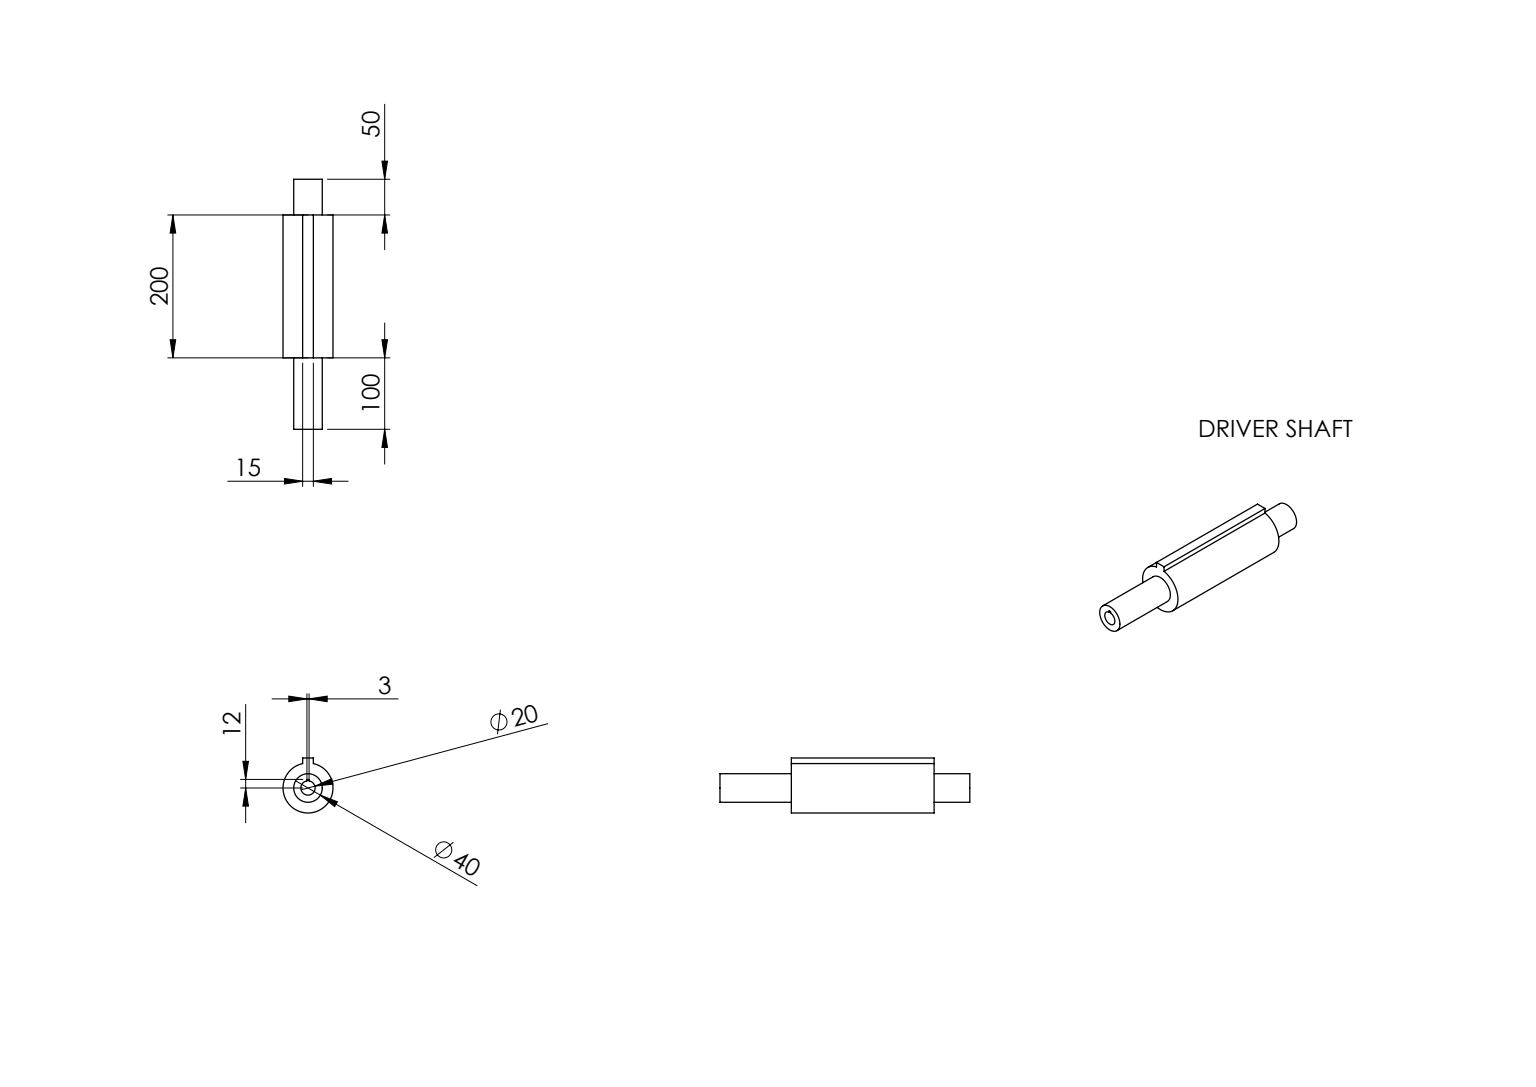
ISO-10303-21;
HEADER;
FILE_DESCRIPTION (('STEP AP214'),
    '1' );
FILE_NAME ('driver shaft.step',
    '2026-10-31T03:46:07',
    ( '' ),
    ( '' ),
    'SwSTEP 2.0',
    'SolidWorks 2026',
    '' );
FILE_SCHEMA (( 'AUTOMOTIVE_DESIGN' ));
ENDSEC;

DATA;
#4=CIRCLE ( 'NONE', #6942, 9.999999999999998224 ) ;
#24=ORIENTED_EDGE ( 'NONE', *, *, #13771, .T. ) ;
#33=DIRECTION ( 'NONE',  ( -1.000000000000000000, -0.000000000000000000, -0.000000000000000000 ) ) ;
#92=DIRECTION ( 'NONE',  ( 1.000000000000000000, 0.000000000000000000, 0.000000000000000000 ) ) ;
#97=ORIENTED_EDGE ( 'NONE', *, *, #11862, .T. ) ;
#125=DIRECTION ( 'NONE',  ( 0.000000000000000000, 0.000000000000000000, 1.000000000000000000 ) ) ;
#141=ORIENTED_EDGE ( 'NONE', *, *, #17752, .T. ) ;
#337=CARTESIAN_POINT ( 'NONE',  ( -2.617478843592795368, -9.739726766683153514, 200.0000120000000265 ) ) ;
#387=LINE ( 'NONE', #18240, #3022 ) ;
#432=CARTESIAN_POINT ( 'NONE',  ( -8.354408924214205001, 5.621797280079010584, 200.0000120000000550 ) ) ;
#474=FACE_OUTER_BOUND ( 'NONE', #7021, .T. ) ;
#545=STYLED_ITEM('',(#23920),#12018);
#550=VERTEX_POINT ( 'NONE', #7568 ) ;
#582=ORIENTED_EDGE ( 'NONE', *, *, #10189, .T. ) ;
#629=VERTEX_POINT ( 'NONE', #2837 ) ;
#663=ORIENTED_EDGE ( 'NONE', *, *, #16433, .T. ) ;
#679=VERTEX_POINT ( 'NONE', #17578 ) ;
#681=CARTESIAN_POINT ( 'NONE',  ( 2.670021022440450587, 9.709363531332249053, 200.0000120000000265 ) ) ;
#699=ORIENTED_EDGE ( 'NONE', *, *, #6704, .F. ) ;
#817=ORIENTED_EDGE ( 'NONE', *, *, #14063, .T. ) ;
#829=VERTEX_POINT ( 'NONE', #1392 ) ;
#869=CARTESIAN_POINT ( 'NONE',  ( -7.499999999999999112, 41.99999999999998579, -100.0000000000000000 ) ) ;
#957=FACE_OUTER_BOUND ( 'NONE', #21689, .T. ) ;
#1000=ORIENTED_EDGE ( 'NONE', *, *, #10407, .F. ) ;
#1015=FACE_OUTER_BOUND ( 'NONE', #12354, .T. ) ;
#1023=VECTOR ( 'NONE', #21634, 1000.000000000000000 ) ;
#1105=DIRECTION ( 'NONE',  ( -0.000000000000000000, -1.000000000000000000, -0.000000000000000000 ) ) ;
#1121=AXIS2_PLACEMENT_3D ( 'NONE', #4909, #12668, #14115 ) ;
#1135=FACE_OUTER_BOUND ( 'NONE', #14500, .T. ) ;
#1144=DIRECTION ( 'NONE',  ( 1.000000000000000000, 0.000000000000000000, 0.000000000000000000 ) ) ;
#1337=ORIENTED_EDGE ( 'NONE', *, *, #20218, .T. ) ;
#1392=CARTESIAN_POINT ( 'NONE',  ( 7.499999999999999112, 41.99999999999998579, -100.0000000000000000 ) ) ;
#1488=CARTESIAN_POINT ( 'NONE',  ( 0.000000000000000000, 0.000000000000000000, 100.0000000000000000 ) ) ;
#1490=DIRECTION ( 'NONE',  ( 0.000000000000000000, -1.000000000000000000, 0.000000000000000000 ) ) ;
#1493=CARTESIAN_POINT ( 'NONE',  ( -7.499999999999999112, 34.18698582794336716, 100.0000000000000000 ) ) ;
#1523=CARTESIAN_POINT ( 'NONE',  ( 0.000000000000000000, 0.000000000000000000, 200.0000119999999981 ) ) ;
#1539=AXIS2_PLACEMENT_3D ( 'NONE', #22452, #8220, #15597 ) ;
#1555=FACE_BOUND ( 'NONE', #9941, .T. ) ;
#1574=EDGE_CURVE ( 'NONE', #629, #10120, #22933, .T. ) ;
#1584=B_SPLINE_CURVE_WITH_KNOTS ( 'NONE', 3,
 ( #12939, #20247, #6002, #2009, #22175, #13293, #18434, #337, #11243, #7702, #11467, #5646, #13054, #14961, #7572, #9399, #3697, #18556 ),
 .UNSPECIFIED., .F., .F.,
 ( 4, 2, 2, 2, 2, 2, 2, 2, 4 ),
 ( 0.5000000000000000000, 0.5625000000000000000, 0.6250000000000001110, 0.6875000000000001110, 0.7500000000000001110, 0.8125000000000001110, 0.8750000000000001110, 0.9375000000000000000, 1.000000000000000000 ),
 .UNSPECIFIED. ) ;
#1642=ADVANCED_FACE ( 'NONE', ( #1555, #7449 ), #14384, .T. ) ;
#1738=ORIENTED_EDGE ( 'NONE', *, *, #15643, .F. ) ;
#1777=EDGE_LOOP ( 'NONE', ( #3273, #11325, #13086, #16443 ) ) ;
#1803=FACE_OUTER_BOUND ( 'NONE', #9769, .T. ) ;
#1880=CARTESIAN_POINT ( 'NONE',  ( 6.811259022622480508, 7.416704320018591368, 200.0000120000000550 ) ) ;
#1932=DIRECTION ( 'NONE',  ( 1.000000000000000000, 0.000000000000000000, -0.000000000000000000 ) ) ;
#1952=ORIENTED_EDGE ( 'NONE', *, *, #22528, .T. ) ;
#1995=CARTESIAN_POINT ( 'NONE',  ( 0.000000000000000000, 0.000000000000000000, 100.0000000000000000 ) ) ;
#1996=VERTEX_POINT ( 'NONE', #23608 ) ;
#2009=CARTESIAN_POINT ( 'NONE',  ( -8.737863883542575039, -5.036189803708990276, 200.0000119999999697 ) ) ;
#2116=ORIENTED_EDGE ( 'NONE', *, *, #20811, .F. ) ;
#2166=EDGE_LOOP ( 'NONE', ( #7941, #3894, #10485, #2701 ) ) ;
#2195=SURFACE_SIDE_STYLE ('',( #4502 ) ) ;
#2221=CARTESIAN_POINT ( 'NONE',  ( -1.500000000000000000, 11.99999999999999822, 200.2421591959677016 ) ) ;
#2225=ADVANCED_FACE ( 'NONE', ( #15529 ), #14083, .F. ) ;
#2257=FACE_BOUND ( 'NONE', #15612, .T. ) ;
#2337=EDGE_CURVE ( 'NONE', #9953, #10712, #15398, .T. ) ;
#2341=SHAPE_REPRESENTATION ( 'driver shaft', ( #11210 ), #22731 ) ;
#2355=PLANE ( 'NONE',  #19619 ) ;
#2381=CARTESIAN_POINT ( 'NONE',  ( 0.000000000000000000, 0.000000000000000000, 150.0000000000000284 ) ) ;
#2384=DIRECTION ( 'NONE',  ( -0.000000000000000000, 1.000000000000000000, 0.000000000000000000 ) ) ;
#2507=UNCERTAINTY_MEASURE_WITH_UNIT (LENGTH_MEASURE( 1.000000000000000082E-05 ), #10014, 'distance_accuracy_value', 'NONE');
#2508=ADVANCED_FACE ( 'NONE', ( #14428 ), #3525, .F. ) ;
#2581=ORIENTED_EDGE ( 'NONE', *, *, #18641, .T. ) ;
#2678=VECTOR ( 'NONE', #22928, 1000.000000000000000 ) ;
#2686=CARTESIAN_POINT ( 'NONE',  ( 1.500000000000000000, 11.99999999999999822, 200.0000000000000000 ) ) ;
#2701=ORIENTED_EDGE ( 'NONE', *, *, #22909, .F. ) ;
#2756=VERTEX_POINT ( 'NONE', #7997 ) ;
#2764=DIRECTION ( 'NONE',  ( 1.000000000000000000, 0.000000000000000000, 0.000000000000000000 ) ) ;
#2814=DIRECTION ( 'NONE',  ( 0.000000000000000000, 0.000000000000000000, 1.000000000000000000 ) ) ;
#2823=DIRECTION ( 'NONE',  ( 0.000000000000000000, 0.000000000000000000, 1.000000000000000000 ) ) ;
#2834=VERTEX_POINT ( 'NONE', #20366 ) ;
#2837=CARTESIAN_POINT ( 'NONE',  ( 20.00000000000000000, 0.000000000000000000, 200.0000000000000000 ) ) ;
#2865=ORIENTED_EDGE ( 'NONE', *, *, #6061, .T. ) ;
#2881=AXIS2_PLACEMENT_3D ( 'NONE', #14839, #8941, #16178 ) ;
#2892=VECTOR ( 'NONE', #19506, 1000.000000000000000 ) ;
#2905=LINE ( 'NONE', #869, #9612 ) ;
#3009=EDGE_CURVE ( 'NONE', #10015, #9003, #20055, .T. ) ;
#3022=VECTOR ( 'NONE', #33, 1000.000000000000000 ) ;
#3025=AXIS2_PLACEMENT_3D ( 'NONE', #2381, #9766, #17122 ) ;
#3050=DIRECTION ( 'NONE',  ( 0.000000000000000000, 0.000000000000000000, -1.000000000000000000 ) ) ;
#3114=DIRECTION ( 'NONE',  ( 0.000000000000000000, 0.000000000000000000, 1.000000000000000000 ) ) ;
#3127=EDGE_CURVE ( 'NONE', #16976, #14993, #12202, .T. ) ;
#3173=ORIENTED_EDGE ( 'NONE', *, *, #8892, .F. ) ;
#3195=FACE_OUTER_BOUND ( 'NONE', #22778, .T. ) ;
#3273=ORIENTED_EDGE ( 'NONE', *, *, #21507, .T. ) ;
#3346=CARTESIAN_POINT ( 'NONE',  ( -3.808014612217195616, 9.322005033491132409, 200.0000120000000550 ) ) ;
#3404=EDGE_CURVE ( 'NONE', #19823, #9902, #4907, .T. ) ;
#3444=VERTEX_POINT ( 'NONE', #19503 ) ;
#3467=DIRECTION ( 'NONE',  ( 0.000000000000000000, 0.000000000000000000, 1.000000000000000000 ) ) ;
#3484=VECTOR ( 'NONE', #7444, 1000.000000000000000 ) ;
#3525=PLANE ( 'NONE',  #22326 ) ;
#3590=PLANE ( 'NONE',  #9679 ) ;
#3697=CARTESIAN_POINT ( 'NONE',  ( 10.00000000000000000, -1.308996938995744097, 200.0000119999999981 ) ) ;
#3712=DIRECTION ( 'NONE',  ( 1.000000000000000000, 0.000000000000000000, 0.000000000000000000 ) ) ;
#3765=ADVANCED_FACE ( 'NONE', ( #21532 ), #13979, .T. ) ;
#3769=DIRECTION ( 'NONE',  ( 1.000000000000000000, 0.000000000000000000, 0.000000000000000000 ) ) ;
#3835=CARTESIAN_POINT ( 'NONE',  ( 0.000000000000000000, 0.000000000000000000, -100.0000000000000000 ) ) ;
#3894=ORIENTED_EDGE ( 'NONE', *, *, #23803, .T. ) ;
#3947=DIRECTION ( 'NONE',  ( -1.000000000000000000, 0.000000000000000000, -0.000000000000000000 ) ) ;
#3955=APPLICATION_CONTEXT ( 'automotive_design' ) ;
#4198=ORIENTED_EDGE ( 'NONE', *, *, #18641, .F. ) ;
#4242=( GEOMETRIC_REPRESENTATION_CONTEXT ( 3 ) GLOBAL_UNCERTAINTY_ASSIGNED_CONTEXT ( ( #19091 ) ) GLOBAL_UNIT_ASSIGNED_CONTEXT ( ( #13364, #6428, #22608 ) ) REPRESENTATION_CONTEXT ( 'NONE', 'WORKASPACE' ) );
#4391=ADVANCED_FACE ( 'NONE', ( #16673 ), #11025, .F. ) ;
#4441=SHAPE_DEFINITION_REPRESENTATION ( #22121, #2341 ) ;
#4502=SURFACE_STYLE_FILL_AREA ( #17191 ) ;
#4519=ORIENTED_EDGE ( 'NONE', *, *, #17042, .F. ) ;
#4550=DIRECTION ( 'NONE',  ( 0.000000000000000000, 0.000000000000000000, -1.000000000000000000 ) ) ;
#4646=CARTESIAN_POINT ( 'NONE',  ( 0.000000000000000000, 0.000000000000000000, -100.0000000000000000 ) ) ;
#4715=ORIENTED_EDGE ( 'NONE', *, *, #2337, .T. ) ;
#4907=LINE ( 'NONE', #8911, #21178 ) ;
#4908=EDGE_LOOP ( 'NONE', ( #8011, #817, #5105, #4519 ) ) ;
#4909=CARTESIAN_POINT ( 'NONE',  ( 1.500000000000000000, 0.000000000000000000, 200.2421591959677016 ) ) ;
#4929=CARTESIAN_POINT ( 'NONE',  ( -20.00000000000000000, 2.449293598294706513E-15, -150.0000000000000000 ) ) ;
#5001=ORIENTED_EDGE ( 'NONE', *, *, #13771, .F. ) ;
#5037=ADVANCED_FACE ( 'NONE', ( #1135 ), #8520, .T. ) ;
#5042=CYLINDRICAL_SURFACE ( 'NONE', #21603, 9.999999999999998224 ) ;
#5052=CARTESIAN_POINT ( 'NONE',  ( 1.500000000000000000, 11.99999999999999822, 150.0000000000000284 ) ) ;
#5065=ORIENTED_EDGE ( 'NONE', *, *, #10407, .T. ) ;
#5105=ORIENTED_EDGE ( 'NONE', *, *, #15119, .T. ) ;
#5108=DIRECTION ( 'NONE',  ( -0.000000000000000000, -0.000000000000000000, -1.000000000000000000 ) ) ;
#5124=CARTESIAN_POINT ( 'NONE',  ( -7.499999999999999112, 34.18698582794336716, 100.0000000000000000 ) ) ;
#5142=ORIENTED_EDGE ( 'NONE', *, *, #3127, .F. ) ;
#5174=CARTESIAN_POINT ( 'NONE',  ( -5.878907051488763358, 8.175524754488199264, 200.0000119999999981 ) ) ;
#5243=CARTESIAN_POINT ( 'NONE',  ( -7.499999999999999112, 34.18698582794336716, 100.0000000000000000 ) ) ;
#5304=DIRECTION ( 'NONE',  ( -0.000000000000000000, -0.000000000000000000, -1.000000000000000000 ) ) ;
#5315=VERTEX_POINT ( 'NONE', #2686 ) ;
#5403=PRODUCT_DEFINITION_FORMATION_WITH_SPECIFIED_SOURCE ( 'ANY', '', #12925, .NOT_KNOWN. ) ;
#5432=CARTESIAN_POINT ( 'NONE',  ( 0.000000000000000000, 0.000000000000000000, 200.0000000000000000 ) ) ;
#5477=LINE ( 'NONE', #12649, #20375 ) ;
#5541=EDGE_LOOP ( 'NONE', ( #2116, #16606, #13467, #12615, #16349, #9301 ) ) ;
#5603=CARTESIAN_POINT ( 'NONE',  ( -1.500000000000000000, 11.99999999999999822, 150.0000000000000284 ) ) ;
#5646=CARTESIAN_POINT ( 'NONE',  ( 5.036189803708990276, -8.737863883542580368, 200.0000119999999981 ) ) ;
#5650=CARTESIAN_POINT ( 'NONE',  ( 0.000000000000000000, 0.000000000000000000, 100.0000000000000000 ) ) ;
#5654=PLANE ( 'NONE',  #5804 ) ;
#5658=LINE ( 'NONE', #13070, #21701 ) ;
#5688=AXIS2_PLACEMENT_3D ( 'NONE', #11158, #8729, #14763 ) ;
#5709=DIRECTION ( 'NONE',  ( 0.000000000000000000, 0.000000000000000000, 1.000000000000000000 ) ) ;
#5735=EDGE_LOOP ( 'NONE', ( #24, #22433, #19438, #15105 ) ) ;
#5747=VECTOR ( 'NONE', #1105, 1000.000000000000000 ) ;
#5761=AXIS2_PLACEMENT_3D ( 'NONE', #16711, #5709, #15386 ) ;
#5771=AXIS2_PLACEMENT_3D ( 'NONE', #7346, #14727, #3712 ) ;
#5775=CARTESIAN_POINT ( 'NONE',  ( 0.000000000000000000, 0.000000000000000000, 200.0000119999999981 ) ) ;
#5804=AXIS2_PLACEMENT_3D ( 'NONE', #16882, #3947, #18926 ) ;
#5848=CARTESIAN_POINT ( 'NONE',  ( 7.499999999999997335, 34.18698582794336005, 100.0000000000000000 ) ) ;
#5872=VECTOR ( 'NONE', #11716, 1000.000000000000000 ) ;
#5915=ADVANCED_FACE ( 'NONE', ( #20144, #16189 ), #3590, .T. ) ;
#5958=ADVANCED_FACE ( 'NONE', ( #2257, #474 ), #17020, .F. ) ;
#5960=CARTESIAN_POINT ( 'NONE',  ( -7.499999999999999112, 41.99999999999998579, -100.0000000000000000 ) ) ;
#5961=ADVANCED_FACE ( 'NONE', ( #20497 ), #5654, .F. ) ;
#6001=CARTESIAN_POINT ( 'NONE',  ( 7.499999999999999112, 41.99999999999998579, 100.0000000000000000 ) ) ;
#6002=CARTESIAN_POINT ( 'NONE',  ( -9.739726766683155290, -2.617478843592798921, 200.0000119999999981 ) ) ;
#6061=EDGE_CURVE ( 'NONE', #2756, #679, #11236, .T. ) ;
#6083=AXIS2_PLACEMENT_3D ( 'NONE', #21310, #2823, #1144 ) ;
#6089=ORIENTED_EDGE ( 'NONE', *, *, #19223, .F. ) ;
#6213=PRODUCT_DEFINITION ( 'UNKNOWN', '', #5403, #9310 ) ;
#6234=DIRECTION ( 'NONE',  ( 0.000000000000000000, -1.000000000000000000, 0.000000000000000000 ) ) ;
#6240=CARTESIAN_POINT ( 'NONE',  ( 9.999999999999998224, 1.224646799147352862E-15, 150.0000000000000284 ) ) ;
#6310=CIRCLE ( 'NONE', #19809, 20.00000000000000000 ) ;
#6312=VERTEX_POINT ( 'NONE', #5052 ) ;
#6322=CARTESIAN_POINT ( 'NONE',  ( -9.999999999999998224, 0.000000000000000000, 200.0000119999999981 ) ) ;
#6412=ORIENTED_EDGE ( 'NONE', *, *, #16214, .F. ) ;
#6428=( NAMED_UNIT ( * ) PLANE_ANGLE_UNIT ( ) SI_UNIT ( $, .RADIAN. ) );
#6454=FACE_OUTER_BOUND ( 'NONE', #5735, .T. ) ;
#6465=LINE ( 'NONE', #12305, #19674 ) ;
#6697=LINE ( 'NONE', #8632, #21508 ) ;
#6704=EDGE_CURVE ( 'NONE', #10742, #8313, #23110, .T. ) ;
#6791=EDGE_LOOP ( 'NONE', ( #11013, #141, #16761, #5142 ) ) ;
#6923=ORIENTED_EDGE ( 'NONE', *, *, #3127, .T. ) ;
#6938=ADVANCED_FACE ( 'NONE', ( #22292 ), #16754, .F. ) ;
#6942=AXIS2_PLACEMENT_3D ( 'NONE', #10985, #3467, #92 ) ;
#7021=EDGE_LOOP ( 'NONE', ( #9205, #5001, #12000, #1000, #17116, #7424 ) ) ;
#7035=CARTESIAN_POINT ( 'NONE',  ( 0.000000000000000000, 0.000000000000000000, 100.0000000000000000 ) ) ;
#7058=EDGE_CURVE ( 'NONE', #15352, #829, #17009, .T. ) ;
#7120=LINE ( 'NONE', #14621, #1023 ) ;
#7146=DIRECTION ( 'NONE',  ( 1.000000000000000000, 0.000000000000000000, 0.000000000000000000 ) ) ;
#7167=CARTESIAN_POINT ( 'NONE',  ( 0.000000000000000000, 0.000000000000000000, -150.0000000000000000 ) ) ;
#7221=CARTESIAN_POINT ( 'NONE',  ( 20.00000000000000000, 0.000000000000000000, -150.0000000000000000 ) ) ;
#7289=DIRECTION ( 'NONE',  ( 0.000000000000000000, 0.000000000000000000, 1.000000000000000000 ) ) ;
#7346=CARTESIAN_POINT ( 'NONE',  ( 0.000000000000000000, 0.000000000000000000, 100.0000000000000000 ) ) ;
#7368=EDGE_LOOP ( 'NONE', ( #10750, #10550 ) ) ;
#7377=EDGE_CURVE ( 'NONE', #2834, #13773, #5658, .T. ) ;
#7424=ORIENTED_EDGE ( 'NONE', *, *, #22404, .F. ) ;
#7441=DIRECTION ( 'NONE',  ( 0.000000000000000000, 0.000000000000000000, 1.000000000000000000 ) ) ;
#7444=DIRECTION ( 'NONE',  ( 0.000000000000000000, 0.000000000000000000, -1.000000000000000000 ) ) ;
#7449=FACE_OUTER_BOUND ( 'NONE', #22066, .T. ) ;
#7456=LINE ( 'NONE', #15207, #21349 ) ;
#7545=VECTOR ( 'NONE', #19872, 1000.000000000000000 ) ;
#7562=CARTESIAN_POINT ( 'NONE',  ( 8.964804008826853021, 4.586179404162092688, 200.0000119999999413 ) ) ;
#7568=CARTESIAN_POINT ( 'NONE',  ( -9.999999999999998224, -6.123233995736763324E-16, 200.0000060000000133 ) ) ;
#7572=CARTESIAN_POINT ( 'NONE',  ( 8.737863883542583920, -5.036189803708986723, 200.0000119999999981 ) ) ;
#7580=DIRECTION ( 'NONE',  ( 0.000000000000000000, 0.000000000000000000, 1.000000000000000000 ) ) ;
#7605=AXIS2_PLACEMENT_3D ( 'NONE', #8929, #7441, #21704 ) ;
#7642=ORIENTED_EDGE ( 'NONE', *, *, #14172, .F. ) ;
#7693=VECTOR ( 'NONE', #7289, 1000.000000000000000 ) ;
#7702=CARTESIAN_POINT ( 'NONE',  ( 1.308996938995748094, -9.999999999999992895, 200.0000120000000265 ) ) ;
#7802=EDGE_CURVE ( 'NONE', #3444, #2834, #14045, .T. ) ;
#7891=( NAMED_UNIT ( * ) SI_UNIT ( $, .STERADIAN. ) SOLID_ANGLE_UNIT ( ) );
#7929=CLOSED_SHELL ( 'NONE', ( #9355, #16700, #15517, #5037, #4391, #14413, #5915, #6938, #17406, #8451, #2225, #20082, #1642, #5958, #2508, #3765, #9150, #19186, #14431, #19939, #5961 ) ) ;
#7941=ORIENTED_EDGE ( 'NONE', *, *, #21647, .T. ) ;
#7972=CARTESIAN_POINT ( 'NONE',  ( 20.00000000000000000, 0.000000000000000000, 100.0000000000000000 ) ) ;
#7997=CARTESIAN_POINT ( 'NONE',  ( -7.499999999999999112, 34.18698582794336716, -100.0000000000000000 ) ) ;
#8007=CIRCLE ( 'NONE', #5688, 20.00000000000000000 ) ;
#8011=ORIENTED_EDGE ( 'NONE', *, *, #20811, .T. ) ;
#8070=FACE_OUTER_BOUND ( 'NONE', #6791, .T. ) ;
#8180=DIRECTION ( 'NONE',  ( 1.000000000000000000, 0.000000000000000000, 0.000000000000000000 ) ) ;
#8220=DIRECTION ( 'NONE',  ( 0.000000000000000000, 0.000000000000000000, 1.000000000000000000 ) ) ;
#8223=CARTESIAN_POINT ( 'NONE',  ( -1.500000000000000000, 11.99999999999999822, 200.2421591959677016 ) ) ;
#8225=CARTESIAN_POINT ( 'NONE',  ( 20.00000000000000000, 0.000000000000000000, -150.0000000000000000 ) ) ;
#8313=VERTEX_POINT ( 'NONE', #8225 ) ;
#8338=PLANE ( 'NONE',  #11091 ) ;
#8371=CARTESIAN_POINT ( 'NONE',  ( 20.00000000000000000, 0.000000000000000000, -100.0000000000000000 ) ) ;
#8427=DIRECTION ( 'NONE',  ( -1.000000000000000000, -0.000000000000000000, 0.000000000000000000 ) ) ;
#8451=ADVANCED_FACE ( 'NONE', ( #957 ), #8338, .F. ) ;
#8468=APPLICATION_CONTEXT ( 'automotive_design' ) ;
#8520=CYLINDRICAL_SURFACE ( 'NONE', #16798, 35.00000000000000000 ) ;
#8543=EDGE_LOOP ( 'NONE', ( #21925, #6923, #97, #11395 ) ) ;
#8564=CARTESIAN_POINT ( 'NONE',  ( -20.00000000000000000, 2.449293598294706513E-15, -100.0000000000000000 ) ) ;
#8632=CARTESIAN_POINT ( 'NONE',  ( 1.500000000000000000, 0.000000000000000000, 150.0000000000000284 ) ) ;
#8650=MECHANICAL_DESIGN_GEOMETRIC_PRESENTATION_REPRESENTATION('',(#545),#20991);
#8729=DIRECTION ( 'NONE',  ( 0.000000000000000000, 0.000000000000000000, 1.000000000000000000 ) ) ;
#8764=CARTESIAN_POINT ( 'NONE',  ( -20.00000000000000000, 2.449293598294706513E-15, -150.0000000000000000 ) ) ;
#8854=ORIENTED_EDGE ( 'NONE', *, *, #14172, .T. ) ;
#8867=CIRCLE ( 'NONE', #5771, 35.00000000000000000 ) ;
#8892=EDGE_CURVE ( 'NONE', #8313, #10742, #19546, .T. ) ;
#8911=CARTESIAN_POINT ( 'NONE',  ( 7.499999999999997335, 34.18698582794336005, 100.0000000000000000 ) ) ;
#8929=CARTESIAN_POINT ( 'NONE',  ( 0.000000000000000000, 0.000000000000000000, -150.0000000000000000 ) ) ;
#8939=FACE_OUTER_BOUND ( 'NONE', #21756, .T. ) ;
#8941=DIRECTION ( 'NONE',  ( 0.000000000000000000, 0.000000000000000000, 1.000000000000000000 ) ) ;
#8942=ORIENTED_EDGE ( 'NONE', *, *, #14743, .T. ) ;
#8975=CYLINDRICAL_SURFACE ( 'NONE', #9968, 35.00000000000000000 ) ;
#9003=VERTEX_POINT ( 'NONE', #6240 ) ;
#9114=VECTOR ( 'NONE', #9843, 1000.000000000000000 ) ;
#9150=ADVANCED_FACE ( 'NONE', ( #1015 ), #22880, .T. ) ;
#9175=ORIENTED_EDGE ( 'NONE', *, *, #20096, .T. ) ;
#9196=PLANE ( 'NONE',  #14654 ) ;
#9205=ORIENTED_EDGE ( 'NONE', *, *, #6061, .F. ) ;
#9283=CARTESIAN_POINT ( 'NONE',  ( 3.808017302909278978, 9.322003897477310730, 200.0000120000000550 ) ) ;
#9301=ORIENTED_EDGE ( 'NONE', *, *, #23613, .F. ) ;
#9310=PRODUCT_DEFINITION_CONTEXT ( 'detailed design', #8468, 'design' ) ;
#9332=CARTESIAN_POINT ( 'NONE',  ( -1.500000000000000000, 11.99999999999999822, 200.0000000000000000 ) ) ;
#9339=CARTESIAN_POINT ( 'NONE',  ( 0.000000000000000000, 0.000000000000000000, 150.0000000000000284 ) ) ;
#9355=ADVANCED_FACE ( 'NONE', ( #10714 ), #23708, .T. ) ;
#9391=CARTESIAN_POINT ( 'NONE',  ( 9.999999999999998224, 6.123233995736764310E-16, 200.0000060000000133 ) ) ;
#9399=CARTESIAN_POINT ( 'NONE',  ( 9.739726766683158843, -2.617478843592797144, 200.0000120000001402 ) ) ;
#9473=CARTESIAN_POINT ( 'NONE',  ( 0.000000000000000000, 0.000000000000000000, 0.000000000000000000 ) ) ;
#9492=DIRECTION ( 'NONE',  ( 1.000000000000000000, 0.000000000000000000, 0.000000000000000000 ) ) ;
#9513=VERTEX_POINT ( 'NONE', #18519 ) ;
#9526=CARTESIAN_POINT ( 'NONE',  ( 0.000000000000000000, 0.000000000000000000, -100.0000000000000000 ) ) ;
#9595=LINE ( 'NONE', #13495, #21994 ) ;
#9609=AXIS2_PLACEMENT_3D ( 'NONE', #5124, #21666, #17924 ) ;
#9612=VECTOR ( 'NONE', #15869, 1000.000000000000000 ) ;
#9638=CIRCLE ( 'NONE', #5761, 35.00000000000000000 ) ;
#9679=AXIS2_PLACEMENT_3D ( 'NONE', #5432, #10766, #12840 ) ;
#9735=DIRECTION ( 'NONE',  ( 0.000000000000000000, 0.000000000000000000, 1.000000000000000000 ) ) ;
#9766=DIRECTION ( 'NONE',  ( 0.000000000000000000, 0.000000000000000000, 1.000000000000000000 ) ) ;
#9769=EDGE_LOOP ( 'NONE', ( #8942, #21106, #12127, #1952, #22281, #17918 ) ) ;
#9808=ORIENTED_EDGE ( 'NONE', *, *, #3009, .F. ) ;
#9843=DIRECTION ( 'NONE',  ( 2.220299922379603824E-16, 1.000000000000000000, 0.000000000000000000 ) ) ;
#9902=VERTEX_POINT ( 'NONE', #11518 ) ;
#9941=EDGE_LOOP ( 'NONE', ( #20109, #11079 ) ) ;
#9953=VERTEX_POINT ( 'NONE', #8564 ) ;
#9957=ORIENTED_EDGE ( 'NONE', *, *, #14183, .T. ) ;
#9968=AXIS2_PLACEMENT_3D ( 'NONE', #7035, #5108, #23684 ) ;
#10002=VECTOR ( 'NONE', #8427, 1000.000000000000000 ) ;
#10014=( LENGTH_UNIT ( ) NAMED_UNIT ( * ) SI_UNIT ( .MILLI., .METRE. ) );
#10015=VERTEX_POINT ( 'NONE', #23164 ) ;
#10043=EDGE_CURVE ( 'NONE', #10742, #9953, #21467, .T. ) ;
#10106=EDGE_CURVE ( 'NONE', #11847, #16299, #20125, .T. ) ;
#10120=VERTEX_POINT ( 'NONE', #21818 ) ;
#10189=EDGE_CURVE ( 'NONE', #1996, #11847, #12337, .T. ) ;
#10243=LINE ( 'NONE', #17584, #2892 ) ;
#10264=CIRCLE ( 'NONE', #23726, 20.00000000000000000 ) ;
#10347=DIRECTION ( 'NONE',  ( 1.000000000000000000, 0.000000000000000000, 0.000000000000000000 ) ) ;
#10359=AXIS2_PLACEMENT_3D ( 'NONE', #7167, #21894, #22024 ) ;
#10362=EDGE_LOOP ( 'NONE', ( #7642, #12187, #1337, #11868 ) ) ;
#10377=CARTESIAN_POINT ( 'NONE',  ( 0.000000000000000000, 11.99999999999999822, 200.0000000000000000 ) ) ;
#10407=EDGE_CURVE ( 'NONE', #9902, #829, #21210, .T. ) ;
#10442=CARTESIAN_POINT ( 'NONE',  ( 35.00000000000000000, 4.286263797015736496E-15, -100.0000000000000000 ) ) ;
#10485=ORIENTED_EDGE ( 'NONE', *, *, #1574, .F. ) ;
#10550=ORIENTED_EDGE ( 'NONE', *, *, #19223, .T. ) ;
#10635=CARTESIAN_POINT ( 'NONE',  ( -1.499999046620369203, 9.887721681869660273, 200.0000060000000133 ) ) ;
#10706=LINE ( 'NONE', #1493, #12551 ) ;
#10712=VERTEX_POINT ( 'NONE', #8371 ) ;
#10714=FACE_OUTER_BOUND ( 'NONE', #2166, .T. ) ;
#10725=DIRECTION ( 'NONE',  ( -1.000000000000000000, 0.000000000000000000, 0.000000000000000000 ) ) ;
#10742=VERTEX_POINT ( 'NONE', #13846 ) ;
#10750=ORIENTED_EDGE ( 'NONE', *, *, #1574, .T. ) ;
#10753=ORIENTED_EDGE ( 'NONE', *, *, #18930, .F. ) ;
#10766=DIRECTION ( 'NONE',  ( 0.000000000000000000, 0.000000000000000000, 1.000000000000000000 ) ) ;
#10871=B_SPLINE_CURVE_WITH_KNOTS ( 'NONE', 3,
 ( #10635, #17974, #3346, #5174, #15288, #432, #15165, #22618, #12935, #20242 ),
 .UNSPECIFIED., .F., .F.,
 ( 4, 2, 2, 2, 4 ),
 ( 0.2739616238528958525, 0.3304712178896719310, 0.3869808119264479540, 0.4434904059632239770, 0.5000000000000000000 ),
 .UNSPECIFIED. ) ;
#10921=AXIS2_PLACEMENT_3D ( 'NONE', #5775, #18431, #18212 ) ;
#10934=DIRECTION ( 'NONE',  ( 0.000000000000000000, 0.000000000000000000, 1.000000000000000000 ) ) ;
#10943=LINE ( 'NONE', #5243, #12734 ) ;
#10985=CARTESIAN_POINT ( 'NONE',  ( 0.000000000000000000, 0.000000000000000000, 150.0000000000000284 ) ) ;
#11013=ORIENTED_EDGE ( 'NONE', *, *, #17522, .T. ) ;
#11022=AXIS2_PLACEMENT_3D ( 'NONE', #11496, #17148, #19059 ) ;
#11025=CYLINDRICAL_SURFACE ( 'NONE', #11022, 9.999999999999998224 ) ;
#11079=ORIENTED_EDGE ( 'NONE', *, *, #11854, .F. ) ;
#11091=AXIS2_PLACEMENT_3D ( 'NONE', #12124, #18449, #16313 ) ;
#11101=CARTESIAN_POINT ( 'NONE',  ( 9.999999999999998224, 1.183533879463814165, 200.0000119999999697 ) ) ;
#11158=CARTESIAN_POINT ( 'NONE',  ( 0.000000000000000000, 0.000000000000000000, 100.0000000000000000 ) ) ;
#11210=AXIS2_PLACEMENT_3D ( 'NONE', #9473, #14914, #3769 ) ;
#11236=CIRCLE ( 'NONE', #13177, 35.00000000000000000 ) ;
#11237=CARTESIAN_POINT ( 'NONE',  ( 1.500000000000000000, 9.886859966642589370, 200.0000119999999981 ) ) ;
#11243=CARTESIAN_POINT ( 'NONE',  ( -1.308996938995744985, -10.00000000000000000, 200.0000119999999697 ) ) ;
#11318=LINE ( 'NONE', #5848, #9114 ) ;
#11325=ORIENTED_EDGE ( 'NONE', *, *, #18716, .F. ) ;
#11395=ORIENTED_EDGE ( 'NONE', *, *, #14063, .F. ) ;
#11412=EDGE_CURVE ( 'NONE', #12624, #3444, #22489, .T. ) ;
#11467=CARTESIAN_POINT ( 'NONE',  ( 2.617478843592798921, -9.739726766683157066, 200.0000119999999981 ) ) ;
#11496=CARTESIAN_POINT ( 'NONE',  ( 0.000000000000000000, 0.000000000000000000, 200.0000119999999981 ) ) ;
#11497=DIRECTION ( 'NONE',  ( 1.000000000000000000, 0.000000000000000000, 0.000000000000000000 ) ) ;
#11518=CARTESIAN_POINT ( 'NONE',  ( 7.499999999999997335, 34.18698582794336005, -100.0000000000000000 ) ) ;
#11658=ORIENTED_EDGE ( 'NONE', *, *, #11412, .F. ) ;
#11673=( LENGTH_UNIT ( ) NAMED_UNIT ( * ) SI_UNIT ( .MILLI., .METRE. ) );
#11682=ORIENTED_EDGE ( 'NONE', *, *, #11412, .T. ) ;
#11716=DIRECTION ( 'NONE',  ( -0.000000000000000000, -0.000000000000000000, -1.000000000000000000 ) ) ;
#11847=VERTEX_POINT ( 'NONE', #18923 ) ;
#11854=EDGE_CURVE ( 'NONE', #15819, #19218, #6310, .T. ) ;
#11862=EDGE_CURVE ( 'NONE', #14993, #15297, #7456, .T. ) ;
#11868=ORIENTED_EDGE ( 'NONE', *, *, #3404, .F. ) ;
#11910=PRESENTATION_STYLE_ASSIGNMENT (( #20805 ) ) ;
#11943=LINE ( 'NONE', #15431, #15422 ) ;
#11999=CARTESIAN_POINT ( 'NONE',  ( 0.000000000000000000, 0.000000000000000000, 200.0000000000000000 ) ) ;
#12000=ORIENTED_EDGE ( 'NONE', *, *, #21507, .F. ) ;
#12018=MANIFOLD_SOLID_BREP ( 'Cut-Extrude-Thin1', #7929 ) ;
#12093=CARTESIAN_POINT ( 'NONE',  ( -1.500000000000000000, 9.886859966642589370, 200.0000119999999981 ) ) ;
#12124=CARTESIAN_POINT ( 'NONE',  ( 7.499999999999997335, 34.18698582794336005, 100.0000000000000000 ) ) ;
#12127=ORIENTED_EDGE ( 'NONE', *, *, #15643, .T. ) ;
#12154=CARTESIAN_POINT ( 'NONE',  ( 7.499999999999999112, 41.99999999999998579, 100.0000000000000000 ) ) ;
#12165=CARTESIAN_POINT ( 'NONE',  ( -7.499999999999999112, 41.99999999999998579, 100.0000000000000000 ) ) ;
#12187=ORIENTED_EDGE ( 'NONE', *, *, #7377, .T. ) ;
#12202=LINE ( 'NONE', #12093, #19275 ) ;
#12222=ORIENTED_EDGE ( 'NONE', *, *, #10043, .T. ) ;
#12305=CARTESIAN_POINT ( 'NONE',  ( -1.500000000000000000, 11.99999999999999822, 150.0000000000000284 ) ) ;
#12337=B_SPLINE_CURVE_WITH_KNOTS ( 'NONE', 3,
 ( #9391, #11101, #20004, #7562, #18421, #1880, #14954, #9283, #681, #15440 ),
 .UNSPECIFIED., .F., .F.,
 ( 4, 2, 2, 2, 4 ),
 ( 0.000000000000000000, 0.05650958017001787154, 0.1130191603400357431, 0.1695287405100536215, 0.2260383206800714861 ),
 .UNSPECIFIED. ) ;
#12354=EDGE_LOOP ( 'NONE', ( #13183, #12419, #19063, #6089 ) ) ;
#12419=ORIENTED_EDGE ( 'NONE', *, *, #11854, .T. ) ;
#12448=ORIENTED_EDGE ( 'NONE', *, *, #7802, .F. ) ;
#12460=LINE ( 'NONE', #10377, #10002 ) ;
#12518=FACE_OUTER_BOUND ( 'NONE', #18348, .T. ) ;
#12551=VECTOR ( 'NONE', #14209, 1000.000000000000000 ) ;
#12615=ORIENTED_EDGE ( 'NONE', *, *, #14183, .F. ) ;
#12624=VERTEX_POINT ( 'NONE', #17890 ) ;
#12649=CARTESIAN_POINT ( 'NONE',  ( 1.500000000000000000, 0.000000000000000000, 200.0000000000000000 ) ) ;
#12668=DIRECTION ( 'NONE',  ( -1.000000000000000000, 0.000000000000000000, -0.000000000000000000 ) ) ;
#12670=CARTESIAN_POINT ( 'NONE',  ( -7.499999999999999112, 41.99999999999998579, 100.0000000000000000 ) ) ;
#12698=EDGE_LOOP ( 'NONE', ( #6412, #582, #18107, #1738 ) ) ;
#12734=VECTOR ( 'NONE', #18265, 1000.000000000000000 ) ;
#12811=CARTESIAN_POINT ( 'NONE',  ( 7.499999999999997335, 34.18698582794336005, 100.0000000000000000 ) ) ;
#12840=DIRECTION ( 'NONE',  ( 1.000000000000000000, 0.000000000000000000, -0.000000000000000000 ) ) ;
#12925=PRODUCT ( 'driver shaft', 'driver shaft', '', ( #21230 ) ) ;
#12935=CARTESIAN_POINT ( 'NONE',  ( -10.00000000000000000, 1.183534169888512011, 200.0000120000000265 ) ) ;
#12939=CARTESIAN_POINT ( 'NONE',  ( -9.999999999999998224, -6.123233995736763324E-16, 200.0000060000000133 ) ) ;
#13015=CARTESIAN_POINT ( 'NONE',  ( 1.500000000000000000, 9.886859966642591147, 150.0000000000000284 ) ) ;
#13054=CARTESIAN_POINT ( 'NONE',  ( 6.145467199749148790, -7.996668423981797780, 200.0000119999999697 ) ) ;
#13070=CARTESIAN_POINT ( 'NONE',  ( 35.00000000000000000, 4.286263797015736496E-15, 100.0000000000000000 ) ) ;
#13086=ORIENTED_EDGE ( 'NONE', *, *, #13936, .F. ) ;
#13177=AXIS2_PLACEMENT_3D ( 'NONE', #9526, #7580, #20371 ) ;
#13183=ORIENTED_EDGE ( 'NONE', *, *, #23803, .F. ) ;
#13208=EDGE_CURVE ( 'NONE', #9513, #12624, #10706, .T. ) ;
#13293=CARTESIAN_POINT ( 'NONE',  ( -6.145467199749147902, -7.996668423981801332, 200.0000120000000265 ) ) ;
#13364=( LENGTH_UNIT ( ) NAMED_UNIT ( * ) SI_UNIT ( .MILLI., .METRE. ) );
#13399=CARTESIAN_POINT ( 'NONE',  ( -1.500000000000000000, 9.886859966642591147, 150.0000000000000284 ) ) ;
#13460=CIRCLE ( 'NONE', #18414, 9.999999999999998224 ) ;
#13467=ORIENTED_EDGE ( 'NONE', *, *, #10189, .F. ) ;
#13495=CARTESIAN_POINT ( 'NONE',  ( -35.00000000000000000, 0.000000000000000000, 100.0000000000000000 ) ) ;
#13610=ORIENTED_EDGE ( 'NONE', *, *, #13208, .T. ) ;
#13637=DIRECTION ( 'NONE',  ( -0.000000000000000000, 1.000000000000000000, 0.000000000000000000 ) ) ;
#13722=FILL_AREA_STYLE_COLOUR ( '', #22355 ) ;
#13771=EDGE_CURVE ( 'NONE', #15265, #2756, #19566, .T. ) ;
#13773=VERTEX_POINT ( 'NONE', #10442 ) ;
#13828=UNCERTAINTY_MEASURE_WITH_UNIT (LENGTH_MEASURE( 1.000000000000000082E-05 ), #11673, 'distance_accuracy_value', 'NONE');
#13844=AXIS2_PLACEMENT_3D ( 'NONE', #21205, #21559, #8180 ) ;
#13846=CARTESIAN_POINT ( 'NONE',  ( -20.00000000000000000, 2.449293598294706513E-15, -150.0000000000000000 ) ) ;
#13854=DIRECTION ( 'NONE',  ( 1.000000000000000000, 0.000000000000000000, 0.000000000000000000 ) ) ;
#13936=EDGE_CURVE ( 'NONE', #15352, #9513, #387, .T. ) ;
#13944=ORIENTED_EDGE ( 'NONE', *, *, #10043, .F. ) ;
#13979=CYLINDRICAL_SURFACE ( 'NONE', #18118, 20.00000000000000000 ) ;
#14045=CIRCLE ( 'NONE', #22091, 35.00000000000000000 ) ;
#14063=EDGE_CURVE ( 'NONE', #21765, #15297, #22576, .T. ) ;
#14083=PLANE ( 'NONE',  #17912 ) ;
#14108=DIRECTION ( 'NONE',  ( 0.000000000000000000, 0.000000000000000000, -1.000000000000000000 ) ) ;
#14115=DIRECTION ( 'NONE',  ( -0.000000000000000000, 0.000000000000000000, 1.000000000000000000 ) ) ;
#14158=DIRECTION ( 'NONE',  ( 0.000000000000000000, 0.000000000000000000, 1.000000000000000000 ) ) ;
#14172=EDGE_CURVE ( 'NONE', #2834, #19823, #8867, .T. ) ;
#14183=EDGE_CURVE ( 'NONE', #550, #1996, #1584, .T. ) ;
#14192=ORIENTED_EDGE ( 'NONE', *, *, #17042, .T. ) ;
#14198=DIRECTION ( 'NONE',  ( 1.000000000000000000, 0.000000000000000000, -0.000000000000000000 ) ) ;
#14209=DIRECTION ( 'NONE',  ( -0.000000000000000000, -1.000000000000000000, -0.000000000000000000 ) ) ;
#14267=DIRECTION ( 'NONE',  ( -0.000000000000000000, -0.000000000000000000, -1.000000000000000000 ) ) ;
#14357=PLANE ( 'NONE',  #1121 ) ;
#14383=ORIENTED_EDGE ( 'NONE', *, *, #8892, .T. ) ;
#14384=PLANE ( 'NONE',  #2881 ) ;
#14413=ADVANCED_FACE ( 'NONE', ( #8070 ), #5042, .F. ) ;
#14428=FACE_OUTER_BOUND ( 'NONE', #19627, .T. ) ;
#14431=ADVANCED_FACE ( 'NONE', ( #3195 ), #14357, .T. ) ;
#14500=EDGE_LOOP ( 'NONE', ( #14625, #12448, #18521, #16118 ) ) ;
#14621=CARTESIAN_POINT ( 'NONE',  ( 1.500000000000000000, 11.99999999999999822, 200.2421591959677016 ) ) ;
#14622=ORIENTED_EDGE ( 'NONE', *, *, #22528, .F. ) ;
#14625=ORIENTED_EDGE ( 'NONE', *, *, #7377, .F. ) ;
#14654=AXIS2_PLACEMENT_3D ( 'NONE', #16556, #20275, #1932 ) ;
#14727=DIRECTION ( 'NONE',  ( 0.000000000000000000, 0.000000000000000000, 1.000000000000000000 ) ) ;
#14743=EDGE_CURVE ( 'NONE', #14993, #10015, #4, .T. ) ;
#14763=DIRECTION ( 'NONE',  ( 1.000000000000000000, 0.000000000000000000, 0.000000000000000000 ) ) ;
#14827=ORIENTED_EDGE ( 'NONE', *, *, #20124, .F. ) ;
#14839=CARTESIAN_POINT ( 'NONE',  ( 0.000000000000000000, 0.000000000000000000, 100.0000000000000000 ) ) ;
#14914=DIRECTION ( 'NONE',  ( 0.000000000000000000, 0.000000000000000000, 1.000000000000000000 ) ) ;
#14954=CARTESIAN_POINT ( 'NONE',  ( 5.878908934339781567, 8.175523358512194250, 200.0000120000000265 ) ) ;
#14961=CARTESIAN_POINT ( 'NONE',  ( 7.996668423981803109, -6.145467199749149678, 200.0000120000000834 ) ) ;
#14993=VERTEX_POINT ( 'NONE', #13399 ) ;
#15066=FACE_OUTER_BOUND ( 'NONE', #4908, .T. ) ;
#15105=ORIENTED_EDGE ( 'NONE', *, *, #18716, .T. ) ;
#15119=EDGE_CURVE ( 'NONE', #15297, #6312, #6465, .T. ) ;
#15165=CARTESIAN_POINT ( 'NONE',  ( -8.964803508279640454, 4.586180457551869871, 200.0000119999999981 ) ) ;
#15207=CARTESIAN_POINT ( 'NONE',  ( -1.500000000000000000, 0.000000000000000000, 150.0000000000000284 ) ) ;
#15231=CARTESIAN_POINT ( 'NONE',  ( 0.000000000000000000, 0.000000000000000000, 100.0000000000000000 ) ) ;
#15265=VERTEX_POINT ( 'NONE', #5960 ) ;
#15274=SHAPE_REPRESENTATION_RELATIONSHIP ( 'NONE' , 'NONE' ,  #2341, #22822 ) ;
#15288=CARTESIAN_POINT ( 'NONE',  ( -6.811257540890722773, 7.416705727137412829, 200.0000120000000265 ) ) ;
#15297=VERTEX_POINT ( 'NONE', #5603 ) ;
#15339=EDGE_CURVE ( 'NONE', #3444, #679, #9595, .T. ) ;
#15352=VERTEX_POINT ( 'NONE', #12154 ) ;
#15386=DIRECTION ( 'NONE',  ( 1.000000000000000000, 0.000000000000000000, 0.000000000000000000 ) ) ;
#15398=CIRCLE ( 'NONE', #19228, 20.00000000000000000 ) ;
#15422=VECTOR ( 'NONE', #6234, 1000.000000000000000 ) ;
#15431=CARTESIAN_POINT ( 'NONE',  ( -1.500000000000000000, 0.000000000000000000, 200.0000000000000000 ) ) ;
#15440=CARTESIAN_POINT ( 'NONE',  ( 1.499998969197076093, 9.887698300110391969, 200.0000060000000133 ) ) ;
#15517=ADVANCED_FACE ( 'NONE', ( #19710 ), #8975, .T. ) ;
#15529=FACE_OUTER_BOUND ( 'NONE', #1777, .T. ) ;
#15597=DIRECTION ( 'NONE',  ( 1.000000000000000000, 0.000000000000000000, 0.000000000000000000 ) ) ;
#15612=EDGE_LOOP ( 'NONE', ( #19078, #4715 ) ) ;
#15643=EDGE_CURVE ( 'NONE', #9003, #16299, #13460, .T. ) ;
#15720=AXIS2_PLACEMENT_3D ( 'NONE', #18100, #14267, #16296 ) ;
#15799=( NAMED_UNIT ( * ) PLANE_ANGLE_UNIT ( ) SI_UNIT ( $, .RADIAN. ) );
#15819=VERTEX_POINT ( 'NONE', #19524 ) ;
#15869=DIRECTION ( 'NONE',  ( -1.000000000000000000, -0.000000000000000000, -0.000000000000000000 ) ) ;
#15911=DIRECTION ( 'NONE',  ( -0.000000000000000000, -0.000000000000000000, -1.000000000000000000 ) ) ;
#15991=LINE ( 'NONE', #6322, #22775 ) ;
#16005=DIRECTION ( 'NONE',  ( -0.000000000000000000, 1.000000000000000000, 0.000000000000000000 ) ) ;
#16118=ORIENTED_EDGE ( 'NONE', *, *, #22404, .T. ) ;
#16178=DIRECTION ( 'NONE',  ( 1.000000000000000000, 0.000000000000000000, -0.000000000000000000 ) ) ;
#16189=FACE_BOUND ( 'NONE', #5541, .T. ) ;
#16214=EDGE_CURVE ( 'NONE', #1996, #9003, #19742, .T. ) ;
#16246=DIRECTION ( 'NONE',  ( -0.000000000000000000, -0.000000000000000000, -1.000000000000000000 ) ) ;
#16296=DIRECTION ( 'NONE',  ( -1.000000000000000000, 0.000000000000000000, 0.000000000000000000 ) ) ;
#16299=VERTEX_POINT ( 'NONE', #13015 ) ;
#16313=DIRECTION ( 'NONE',  ( -2.220299922379604070E-16, -1.000000000000000000, 0.000000000000000000 ) ) ;
#16349=ORIENTED_EDGE ( 'NONE', *, *, #17522, .F. ) ;
#16413=ORIENTED_EDGE ( 'NONE', *, *, #13936, .T. ) ;
#16433=EDGE_CURVE ( 'NONE', #19823, #15352, #11318, .T. ) ;
#16443=ORIENTED_EDGE ( 'NONE', *, *, #7058, .T. ) ;
#16556=CARTESIAN_POINT ( 'NONE',  ( 0.000000000000000000, 0.000000000000000000, 150.0000000000000284 ) ) ;
#16585=CARTESIAN_POINT ( 'NONE',  ( 0.000000000000000000, 0.000000000000000000, -150.0000000000000000 ) ) ;
#16606=ORIENTED_EDGE ( 'NONE', *, *, #20124, .T. ) ;
#16616=VECTOR ( 'NONE', #14158, 1000.000000000000000 ) ;
#16659=ORIENTED_EDGE ( 'NONE', *, *, #2337, .F. ) ;
#16673=FACE_OUTER_BOUND ( 'NONE', #17163, .T. ) ;
#16700=ADVANCED_FACE ( 'NONE', ( #12518 ), #21764, .T. ) ;
#16711=CARTESIAN_POINT ( 'NONE',  ( 0.000000000000000000, 0.000000000000000000, -100.0000000000000000 ) ) ;
#16754=CYLINDRICAL_SURFACE ( 'NONE', #10921, 9.999999999999998224 ) ;
#16761=ORIENTED_EDGE ( 'NONE', *, *, #14743, .F. ) ;
#16798=AXIS2_PLACEMENT_3D ( 'NONE', #1488, #16246, #23347 ) ;
#16876=DIRECTION ( 'NONE',  ( 1.000000000000000000, 0.000000000000000000, 0.000000000000000000 ) ) ;
#16882=CARTESIAN_POINT ( 'NONE',  ( -1.500000000000000000, 0.000000000000000000, 200.2421591959677016 ) ) ;
#16923=ORIENTED_EDGE ( 'NONE', *, *, #3404, .T. ) ;
#16976=VERTEX_POINT ( 'NONE', #18229 ) ;
#17000=AXIS2_PLACEMENT_3D ( 'NONE', #3835, #17127, #20872 ) ;
#17009=LINE ( 'NONE', #6001, #5872 ) ;
#17020=PLANE ( 'NONE',  #17000 ) ;
#17042=EDGE_CURVE ( 'NONE', #5315, #6312, #7120, .T. ) ;
#17102=DIRECTION ( 'NONE',  ( 0.000000000000000000, 0.000000000000000000, 1.000000000000000000 ) ) ;
#17114=AXIS2_PLACEMENT_3D ( 'NONE', #15231, #125, #11497 ) ;
#17116=ORIENTED_EDGE ( 'NONE', *, *, #20218, .F. ) ;
#17122=DIRECTION ( 'NONE',  ( 1.000000000000000000, 0.000000000000000000, 0.000000000000000000 ) ) ;
#17127=DIRECTION ( 'NONE',  ( 0.000000000000000000, 0.000000000000000000, 1.000000000000000000 ) ) ;
#17148=DIRECTION ( 'NONE',  ( 0.000000000000000000, 0.000000000000000000, -1.000000000000000000 ) ) ;
#17163=EDGE_LOOP ( 'NONE', ( #9957, #17421, #9808, #19739 ) ) ;
#17191=FILL_AREA_STYLE ('',( #13722 ) ) ;
#17294=ORIENTED_EDGE ( 'NONE', *, *, #7058, .F. ) ;
#17406=ADVANCED_FACE ( 'NONE', ( #8939 ), #23402, .T. ) ;
#17421=ORIENTED_EDGE ( 'NONE', *, *, #16214, .T. ) ;
#17522=EDGE_CURVE ( 'NONE', #16976, #550, #10871, .T. ) ;
#17576=CARTESIAN_POINT ( 'NONE',  ( 9.999999999999998224, 1.224646799147352862E-15, 200.0000119999999981 ) ) ;
#17578=CARTESIAN_POINT ( 'NONE',  ( -35.00000000000000000, 0.000000000000000000, -100.0000000000000000 ) ) ;
#17584=CARTESIAN_POINT ( 'NONE',  ( 20.00000000000000000, 0.000000000000000000, -150.0000000000000000 ) ) ;
#17642=CIRCLE ( 'NONE', #6083, 35.00000000000000000 ) ;
#17752=EDGE_CURVE ( 'NONE', #550, #10015, #15991, .T. ) ;
#17823=CARTESIAN_POINT ( 'NONE',  ( 7.499999999999997335, 34.18698582794336005, -100.0000000000000000 ) ) ;
#17890=CARTESIAN_POINT ( 'NONE',  ( -7.499999999999999112, 34.18698582794336716, 100.0000000000000000 ) ) ;
#17912=AXIS2_PLACEMENT_3D ( 'NONE', #12165, #22751, #21181 ) ;
#17913=CARTESIAN_POINT ( 'NONE',  ( 0.000000000000000000, 0.000000000000000000, -150.0000000000000000 ) ) ;
#17914=DIRECTION ( 'NONE',  ( 0.000000000000000000, 0.000000000000000000, 1.000000000000000000 ) ) ;
#17918=ORIENTED_EDGE ( 'NONE', *, *, #11862, .F. ) ;
#17924=DIRECTION ( 'NONE',  ( 0.000000000000000000, 0.000000000000000000, -1.000000000000000000 ) ) ;
#17974=CARTESIAN_POINT ( 'NONE',  ( -2.670017925772866452, 9.709364418299751165, 200.0000120000000265 ) ) ;
#18100=CARTESIAN_POINT ( 'NONE',  ( 0.000000000000000000, 0.000000000000000000, 100.0000000000000000 ) ) ;
#18107=ORIENTED_EDGE ( 'NONE', *, *, #10106, .T. ) ;
#18118=AXIS2_PLACEMENT_3D ( 'NONE', #23101, #17914, #21412 ) ;
#18212=DIRECTION ( 'NONE',  ( -1.000000000000000000, 0.000000000000000000, 0.000000000000000000 ) ) ;
#18229=CARTESIAN_POINT ( 'NONE',  ( -1.499999046620369203, 9.887721681869660273, 200.0000060000000133 ) ) ;
#18240=CARTESIAN_POINT ( 'NONE',  ( -7.499999999999999112, 41.99999999999998579, 100.0000000000000000 ) ) ;
#18265=DIRECTION ( 'NONE',  ( -0.000000000000000000, -0.000000000000000000, -1.000000000000000000 ) ) ;
#18348=EDGE_LOOP ( 'NONE', ( #14383, #12222, #10753, #4198 ) ) ;
#18414=AXIS2_PLACEMENT_3D ( 'NONE', #9339, #20652, #18834 ) ;
#18421=CARTESIAN_POINT ( 'NONE',  ( 8.354409714504226869, 5.621796044507131107, 200.0000120000000265 ) ) ;
#18431=DIRECTION ( 'NONE',  ( 0.000000000000000000, 0.000000000000000000, -1.000000000000000000 ) ) ;
#18434=CARTESIAN_POINT ( 'NONE',  ( -5.036189803708989388, -8.737863883542578591, 200.0000120000000265 ) ) ;
#18449=DIRECTION ( 'NONE',  ( -1.000000000000000000, 2.220299922379604070E-16, 0.000000000000000000 ) ) ;
#18481=DIRECTION ( 'NONE',  ( 0.000000000000000000, 0.000000000000000000, 1.000000000000000000 ) ) ;
#18491=CIRCLE ( 'NONE', #1539, 20.00000000000000000 ) ;
#18519=CARTESIAN_POINT ( 'NONE',  ( -7.499999999999999112, 41.99999999999998579, 100.0000000000000000 ) ) ;
#18521=ORIENTED_EDGE ( 'NONE', *, *, #15339, .T. ) ;
#18556=CARTESIAN_POINT ( 'NONE',  ( 9.999999999999998224, 6.123233995736764310E-16, 200.0000060000000133 ) ) ;
#18609=ORIENTED_EDGE ( 'NONE', *, *, #16433, .F. ) ;
#18641=EDGE_CURVE ( 'NONE', #8313, #10712, #10243, .T. ) ;
#18716=EDGE_CURVE ( 'NONE', #9513, #15265, #21799, .T. ) ;
#18766=DIRECTION ( 'NONE',  ( 1.000000000000000000, 0.000000000000000000, 0.000000000000000000 ) ) ;
#18834=DIRECTION ( 'NONE',  ( 1.000000000000000000, 0.000000000000000000, 0.000000000000000000 ) ) ;
#18864=AXIS2_PLACEMENT_3D ( 'NONE', #20406, #18481, #20166 ) ;
#18923=CARTESIAN_POINT ( 'NONE',  ( 1.499998969197076093, 9.887698300110391969, 200.0000060000000133 ) ) ;
#18926=DIRECTION ( 'NONE',  ( -0.000000000000000000, 0.000000000000000000, 1.000000000000000000 ) ) ;
#18930=EDGE_CURVE ( 'NONE', #10712, #9953, #10264, .T. ) ;
#18999=CARTESIAN_POINT ( 'NONE',  ( 0.000000000000000000, 0.000000000000000000, -100.0000000000000000 ) ) ;
#19059=DIRECTION ( 'NONE',  ( -1.000000000000000000, 0.000000000000000000, 0.000000000000000000 ) ) ;
#19063=ORIENTED_EDGE ( 'NONE', *, *, #22909, .T. ) ;
#19078=ORIENTED_EDGE ( 'NONE', *, *, #18930, .T. ) ;
#19091=UNCERTAINTY_MEASURE_WITH_UNIT (LENGTH_MEASURE( 1.000000000000000082E-05 ), #13364, 'distance_accuracy_value', 'NONE');
#19152=( NAMED_UNIT ( * ) SI_UNIT ( $, .STERADIAN. ) SOLID_ANGLE_UNIT ( ) );
#19186=ADVANCED_FACE ( 'NONE', ( #1803 ), #9196, .T. ) ;
#19218=VERTEX_POINT ( 'NONE', #7972 ) ;
#19223=EDGE_CURVE ( 'NONE', #10120, #629, #18491, .T. ) ;
#19228=AXIS2_PLACEMENT_3D ( 'NONE', #4646, #2814, #13854 ) ;
#19264=DIRECTION ( 'NONE',  ( 2.220299922379603824E-16, 1.000000000000000000, 0.000000000000000000 ) ) ;
#19268=STYLED_ITEM ( 'NONE', ( #11910 ), #22822 ) ;
#19275=VECTOR ( 'NONE', #4550, 1000.000000000000000 ) ;
#19304=DIRECTION ( 'NONE',  ( 0.000000000000000000, 0.000000000000000000, 1.000000000000000000 ) ) ;
#19438=ORIENTED_EDGE ( 'NONE', *, *, #13208, .F. ) ;
#19503=CARTESIAN_POINT ( 'NONE',  ( -35.00000000000000000, 0.000000000000000000, 100.0000000000000000 ) ) ;
#19506=DIRECTION ( 'NONE',  ( 0.000000000000000000, 0.000000000000000000, 1.000000000000000000 ) ) ;
#19524=CARTESIAN_POINT ( 'NONE',  ( -20.00000000000000000, 2.449293598294706513E-15, 100.0000000000000000 ) ) ;
#19546=CIRCLE ( 'NONE', #7605, 20.00000000000000000 ) ;
#19566=LINE ( 'NONE', #23439, #5747 ) ;
#19598=EDGE_LOOP ( 'NONE', ( #13944, #21694, #2581, #16659 ) ) ;
#19619=AXIS2_PLACEMENT_3D ( 'NONE', #2221, #13637, #22398 ) ;
#19627=EDGE_LOOP ( 'NONE', ( #3173, #699 ) ) ;
#19674=VECTOR ( 'NONE', #10347, 1000.000000000000000 ) ;
#19710=FACE_OUTER_BOUND ( 'NONE', #10362, .T. ) ;
#19731=LINE ( 'NONE', #8764, #7693 ) ;
#19739=ORIENTED_EDGE ( 'NONE', *, *, #17752, .F. ) ;
#19742=LINE ( 'NONE', #17576, #20360 ) ;
#19809=AXIS2_PLACEMENT_3D ( 'NONE', #5650, #20493, #16876 ) ;
#19823=VERTEX_POINT ( 'NONE', #12811 ) ;
#19872=DIRECTION ( 'NONE',  ( -0.000000000000000000, -0.000000000000000000, -1.000000000000000000 ) ) ;
#19912=LINE ( 'NONE', #7221, #16616 ) ;
#19939=ADVANCED_FACE ( 'NONE', ( #15066 ), #2355, .F. ) ;
#19982=ORIENTED_EDGE ( 'NONE', *, *, #7802, .T. ) ;
#20004=CARTESIAN_POINT ( 'NONE',  ( 9.787707486204086038, 2.366756136221725981, 200.0000120000000265 ) ) ;
#20055=CIRCLE ( 'NONE', #3025, 9.999999999999998224 ) ;
#20082=ADVANCED_FACE ( 'NONE', ( #6454 ), #22017, .F. ) ;
#20096=EDGE_CURVE ( 'NONE', #12624, #2756, #10943, .T. ) ;
#20109=ORIENTED_EDGE ( 'NONE', *, *, #21647, .F. ) ;
#20124=EDGE_CURVE ( 'NONE', #5315, #11847, #5477, .T. ) ;
#20125=LINE ( 'NONE', #11237, #3484 ) ;
#20144=FACE_OUTER_BOUND ( 'NONE', #7368, .T. ) ;
#20166=DIRECTION ( 'NONE',  ( 1.000000000000000000, 0.000000000000000000, 0.000000000000000000 ) ) ;
#20218=EDGE_CURVE ( 'NONE', #13773, #9902, #9638, .T. ) ;
#20242=CARTESIAN_POINT ( 'NONE',  ( -9.999999999999998224, -6.123233995736763324E-16, 200.0000060000000133 ) ) ;
#20247=CARTESIAN_POINT ( 'NONE',  ( -10.00000000000000178, -1.308996938995748760, 200.0000120000000550 ) ) ;
#20275=DIRECTION ( 'NONE',  ( 0.000000000000000000, 0.000000000000000000, 1.000000000000000000 ) ) ;
#20360=VECTOR ( 'NONE', #14108, 1000.000000000000000 ) ;
#20366=CARTESIAN_POINT ( 'NONE',  ( 35.00000000000000000, 4.286263797015736496E-15, 100.0000000000000000 ) ) ;
#20371=DIRECTION ( 'NONE',  ( 1.000000000000000000, 0.000000000000000000, 0.000000000000000000 ) ) ;
#20375=VECTOR ( 'NONE', #1490, 1000.000000000000000 ) ;
#20406=CARTESIAN_POINT ( 'NONE',  ( 0.000000000000000000, 0.000000000000000000, -150.0000000000000000 ) ) ;
#20439=VECTOR ( 'NONE', #3114, 1000.000000000000000 ) ;
#20493=DIRECTION ( 'NONE',  ( 0.000000000000000000, 0.000000000000000000, 1.000000000000000000 ) ) ;
#20497=FACE_OUTER_BOUND ( 'NONE', #8543, .T. ) ;
#20623=AXIS2_PLACEMENT_3D ( 'NONE', #11999, #19304, #2764 ) ;
#20652=DIRECTION ( 'NONE',  ( 0.000000000000000000, 0.000000000000000000, 1.000000000000000000 ) ) ;
#20680=DIRECTION ( 'NONE',  ( -0.000000000000000000, -0.000000000000000000, -1.000000000000000000 ) ) ;
#20805=SURFACE_STYLE_USAGE ( .BOTH. , #2195 ) ;
#20811=EDGE_CURVE ( 'NONE', #5315, #21765, #12460, .T. ) ;
#20872=DIRECTION ( 'NONE',  ( 1.000000000000000000, 0.000000000000000000, -0.000000000000000000 ) ) ;
#20991=( GEOMETRIC_REPRESENTATION_CONTEXT ( 3 ) GLOBAL_UNCERTAINTY_ASSIGNED_CONTEXT ( ( #2507 ) ) GLOBAL_UNIT_ASSIGNED_CONTEXT ( ( #10014, #15799, #19152 ) ) REPRESENTATION_CONTEXT ( 'NONE', 'WORKASPACE' ) );
#21042=( NAMED_UNIT ( * ) PLANE_ANGLE_UNIT ( ) SI_UNIT ( $, .RADIAN. ) );
#21085=AXIS2_PLACEMENT_3D ( 'NONE', #16585, #23802, #7146 ) ;
#21106=ORIENTED_EDGE ( 'NONE', *, *, #3009, .T. ) ;
#21178=VECTOR ( 'NONE', #15911, 1000.000000000000000 ) ;
#21181=DIRECTION ( 'NONE',  ( 0.000000000000000000, -0.000000000000000000, -1.000000000000000000 ) ) ;
#21205=CARTESIAN_POINT ( 'NONE',  ( 0.000000000000000000, 0.000000000000000000, -150.0000000000000000 ) ) ;
#21210=LINE ( 'NONE', #17823, #23543 ) ;
#21230=PRODUCT_CONTEXT ( 'NONE', #3955, 'mechanical' ) ;
#21310=CARTESIAN_POINT ( 'NONE',  ( 0.000000000000000000, 0.000000000000000000, -100.0000000000000000 ) ) ;
#21349=VECTOR ( 'NONE', #2384, 1000.000000000000000 ) ;
#21412=DIRECTION ( 'NONE',  ( 1.000000000000000000, 0.000000000000000000, 0.000000000000000000 ) ) ;
#21448=ORIENTED_EDGE ( 'NONE', *, *, #15339, .F. ) ;
#21467=LINE ( 'NONE', #4929, #20439 ) ;
#21507=EDGE_CURVE ( 'NONE', #829, #15265, #2905, .T. ) ;
#21508=VECTOR ( 'NONE', #16005, 1000.000000000000000 ) ;
#21532=FACE_OUTER_BOUND ( 'NONE', #19598, .T. ) ;
#21559=DIRECTION ( 'NONE',  ( 0.000000000000000000, 0.000000000000000000, 1.000000000000000000 ) ) ;
#21603=AXIS2_PLACEMENT_3D ( 'NONE', #1523, #23375, #10725 ) ;
#21634=DIRECTION ( 'NONE',  ( 0.000000000000000000, 0.000000000000000000, -1.000000000000000000 ) ) ;
#21647=EDGE_CURVE ( 'NONE', #19218, #15819, #8007, .T. ) ;
#21666=DIRECTION ( 'NONE',  ( 1.000000000000000000, 0.000000000000000000, 0.000000000000000000 ) ) ;
#21689=EDGE_LOOP ( 'NONE', ( #5065, #17294, #18609, #16923 ) ) ;
#21694=ORIENTED_EDGE ( 'NONE', *, *, #6704, .T. ) ;
#21701=VECTOR ( 'NONE', #5304, 1000.000000000000000 ) ;
#21704=DIRECTION ( 'NONE',  ( 1.000000000000000000, 0.000000000000000000, 0.000000000000000000 ) ) ;
#21756=EDGE_LOOP ( 'NONE', ( #21448, #11658, #9175, #2865 ) ) ;
#21764=CYLINDRICAL_SURFACE ( 'NONE', #21085, 20.00000000000000000 ) ;
#21765=VERTEX_POINT ( 'NONE', #9332 ) ;
#21799=LINE ( 'NONE', #12670, #7545 ) ;
#21818=CARTESIAN_POINT ( 'NONE',  ( -20.00000000000000000, 2.449293598294706513E-15, 200.0000000000000000 ) ) ;
#21894=DIRECTION ( 'NONE',  ( 0.000000000000000000, 0.000000000000000000, 1.000000000000000000 ) ) ;
#21925=ORIENTED_EDGE ( 'NONE', *, *, #23613, .T. ) ;
#21994=VECTOR ( 'NONE', #20680, 1000.000000000000000 ) ;
#22017=PLANE ( 'NONE',  #9609 ) ;
#22024=DIRECTION ( 'NONE',  ( 1.000000000000000000, 0.000000000000000000, 0.000000000000000000 ) ) ;
#22066=EDGE_LOOP ( 'NONE', ( #11682, #19982, #8854, #663, #16413, #13610 ) ) ;
#22091=AXIS2_PLACEMENT_3D ( 'NONE', #1995, #17102, #18766 ) ;
#22104=ORIENTED_EDGE ( 'NONE', *, *, #10106, .F. ) ;
#22121=PRODUCT_DEFINITION_SHAPE ( 'NONE', 'NONE',  #6213 ) ;
#22175=CARTESIAN_POINT ( 'NONE',  ( -7.996668423981801332, -6.145467199749147902, 200.0000120000000265 ) ) ;
#22281=ORIENTED_EDGE ( 'NONE', *, *, #15119, .F. ) ;
#22292=FACE_OUTER_BOUND ( 'NONE', #12698, .T. ) ;
#22326=AXIS2_PLACEMENT_3D ( 'NONE', #17913, #10934, #14198 ) ;
#22355=COLOUR_RGB ( '',0.8941176470588234615, 0.8941176470588234615, 0.8941176470588234615 ) ;
#22398=DIRECTION ( 'NONE',  ( 0.000000000000000000, -0.000000000000000000, 1.000000000000000000 ) ) ;
#22404=EDGE_CURVE ( 'NONE', #679, #13773, #17642, .T. ) ;
#22433=ORIENTED_EDGE ( 'NONE', *, *, #20096, .F. ) ;
#22452=CARTESIAN_POINT ( 'NONE',  ( 0.000000000000000000, 0.000000000000000000, 200.0000000000000000 ) ) ;
#22489=CIRCLE ( 'NONE', #17114, 35.00000000000000000 ) ;
#22528=EDGE_CURVE ( 'NONE', #16299, #6312, #6697, .T. ) ;
#22576=LINE ( 'NONE', #8223, #2678 ) ;
#22608=( NAMED_UNIT ( * ) SI_UNIT ( $, .STERADIAN. ) SOLID_ANGLE_UNIT ( ) );
#22618=CARTESIAN_POINT ( 'NONE',  ( -9.787707380959941972, 2.366756716689722317, 200.0000119999999697 ) ) ;
#22731=( GEOMETRIC_REPRESENTATION_CONTEXT ( 3 ) GLOBAL_UNCERTAINTY_ASSIGNED_CONTEXT ( ( #13828 ) ) GLOBAL_UNIT_ASSIGNED_CONTEXT ( ( #11673, #21042, #7891 ) ) REPRESENTATION_CONTEXT ( 'NONE', 'WORKASPACE' ) );
#22751=DIRECTION ( 'NONE',  ( 0.000000000000000000, -1.000000000000000000, 0.000000000000000000 ) ) ;
#22775=VECTOR ( 'NONE', #3050, 1000.000000000000000 ) ;
#22778=EDGE_LOOP ( 'NONE', ( #14192, #14622, #22104, #14827 ) ) ;
#22822=ADVANCED_BREP_SHAPE_REPRESENTATION ( '', ( #12018, #11210 ), #22731 ) ;
#22880=CYLINDRICAL_SURFACE ( 'NONE', #13844, 20.00000000000000000 ) ;
#22909=EDGE_CURVE ( 'NONE', #19218, #629, #19912, .T. ) ;
#22928=DIRECTION ( 'NONE',  ( 0.000000000000000000, 0.000000000000000000, -1.000000000000000000 ) ) ;
#22933=CIRCLE ( 'NONE', #20623, 20.00000000000000000 ) ;
#23101=CARTESIAN_POINT ( 'NONE',  ( 0.000000000000000000, 0.000000000000000000, -150.0000000000000000 ) ) ;
#23110=CIRCLE ( 'NONE', #18864, 20.00000000000000000 ) ;
#23131=MECHANICAL_DESIGN_GEOMETRIC_PRESENTATION_REPRESENTATION('',(#19268),#4242);
#23164=CARTESIAN_POINT ( 'NONE',  ( -9.999999999999998224, 0.000000000000000000, 150.0000000000000284 ) ) ;
#23347=DIRECTION ( 'NONE',  ( -1.000000000000000000, 0.000000000000000000, 0.000000000000000000 ) ) ;
#23375=DIRECTION ( 'NONE',  ( 0.000000000000000000, 0.000000000000000000, -1.000000000000000000 ) ) ;
#23402=CYLINDRICAL_SURFACE ( 'NONE', #15720, 35.00000000000000000 ) ;
#23439=CARTESIAN_POINT ( 'NONE',  ( -7.499999999999999112, 34.18698582794336716, -100.0000000000000000 ) ) ;
#23543=VECTOR ( 'NONE', #19264, 1000.000000000000000 ) ;
#23608=CARTESIAN_POINT ( 'NONE',  ( 9.999999999999998224, 6.123233995736764310E-16, 200.0000060000000133 ) ) ;
#23613=EDGE_CURVE ( 'NONE', #21765, #16976, #11943, .T. ) ;
#23684=DIRECTION ( 'NONE',  ( -1.000000000000000000, 0.000000000000000000, 0.000000000000000000 ) ) ;
#23708=CYLINDRICAL_SURFACE ( 'NONE', #10359, 20.00000000000000000 ) ;
#23726=AXIS2_PLACEMENT_3D ( 'NONE', #18999, #9735, #9492 ) ;
#23802=DIRECTION ( 'NONE',  ( 0.000000000000000000, 0.000000000000000000, 1.000000000000000000 ) ) ;
#23803=EDGE_CURVE ( 'NONE', #15819, #10120, #19731, .T. ) ;
#23914=COLOUR_RGB('Grey',0.48,0.52,0.57);
#23915=FILL_AREA_STYLE_COLOUR('',#23914);
#23916=FILL_AREA_STYLE('',(#23915));
#23917=SURFACE_STYLE_FILL_AREA(#23916);
#23918=SURFACE_SIDE_STYLE('',(#23917));
#23919=SURFACE_STYLE_USAGE(.BOTH.,#23918);
#23920=PRESENTATION_STYLE_ASSIGNMENT((#23919));
ENDSEC;
END-ISO-10303-21;
